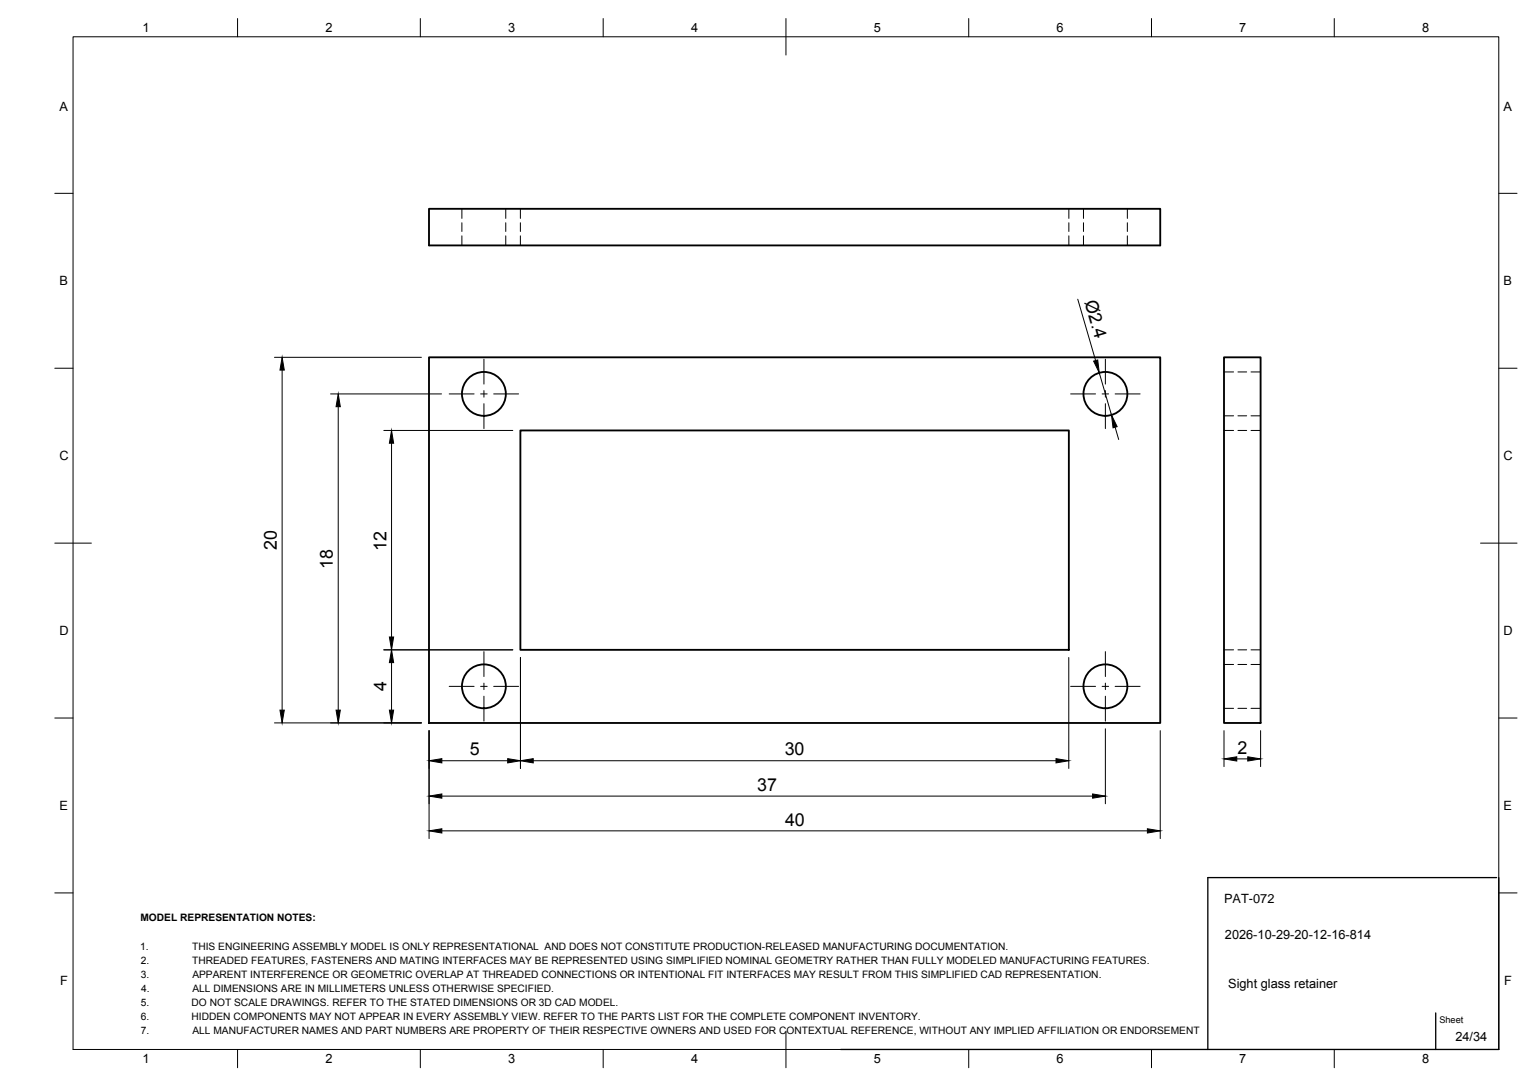
ISO-10303-21;
HEADER;
/* Generated by software containing ST-Developer
 * from STEP Tools, Inc. (www.steptools.com) 
 */

FILE_DESCRIPTION(
/* description */ ('PAT-072'),
/* implementation_level */ '2;1');

FILE_NAME(
/* name */ 'Sight glass retainer.step',
/* time_stamp */ '2026-10-29T20:11:56-07:00',
/* author */ (''),
/* organization */ (''),
/* preprocessor_version */ 'ST-DEVELOPER v20.2',
/* originating_system */ 'Autodesk Translation Framework v15.17.0.0',
/* authorisation */ '');

FILE_SCHEMA (('AUTOMOTIVE_DESIGN { 1 0 10303 214 3 1 1 }'));
ENDSEC;

DATA;
#10=MECHANICAL_DESIGN_GEOMETRIC_PRESENTATION_REPRESENTATION('',(#353),#11432);
#281=SHAPE_REPRESENTATION_RELATIONSHIP('SRR','None',#11585,#317);
#317=ADVANCED_BREP_SHAPE_REPRESENTATION('',(#389),#11416);
#353=STYLED_ITEM('',(#11812),#389);
#389=MANIFOLD_SOLID_BREP('Body1',#6088);
#518=FACE_BOUND('',#1510,.T.);
#519=FACE_BOUND('',#1511,.T.);
#520=FACE_BOUND('',#1512,.T.);
#521=FACE_BOUND('',#1513,.T.);
#522=FACE_BOUND('',#1514,.T.);
#523=FACE_BOUND('',#1517,.T.);
#524=FACE_BOUND('',#1518,.T.);
#525=FACE_BOUND('',#1519,.T.);
#526=FACE_BOUND('',#1520,.T.);
#527=FACE_BOUND('',#1521,.T.);
#692=PLANE('',#6942);
#693=PLANE('',#6943);
#694=PLANE('',#6944);
#695=PLANE('',#6945);
#696=PLANE('',#6946);
#697=PLANE('',#6947);
#698=PLANE('',#6948);
#699=PLANE('',#6949);
#700=PLANE('',#6950);
#701=PLANE('',#6951);
#1013=FACE_OUTER_BOUND('',#1501,.T.);
#1014=FACE_OUTER_BOUND('',#1502,.T.);
#1015=FACE_OUTER_BOUND('',#1503,.T.);
#1016=FACE_OUTER_BOUND('',#1504,.T.);
#1017=FACE_OUTER_BOUND('',#1505,.T.);
#1018=FACE_OUTER_BOUND('',#1506,.T.);
#1019=FACE_OUTER_BOUND('',#1507,.T.);
#1020=FACE_OUTER_BOUND('',#1508,.T.);
#1021=FACE_OUTER_BOUND('',#1509,.T.);
#1022=FACE_OUTER_BOUND('',#1515,.T.);
#1023=FACE_OUTER_BOUND('',#1516,.T.);
#1024=FACE_OUTER_BOUND('',#1522,.T.);
#1025=FACE_OUTER_BOUND('',#1523,.T.);
#1026=FACE_OUTER_BOUND('',#1524,.T.);
#1501=EDGE_LOOP('',(#4934,#4935,#4936,#4937));
#1502=EDGE_LOOP('',(#4938,#4939,#4940,#4941));
#1503=EDGE_LOOP('',(#4942,#4943,#4944,#4945));
#1504=EDGE_LOOP('',(#4946,#4947,#4948,#4949));
#1505=EDGE_LOOP('',(#4950,#4951,#4952,#4953));
#1506=EDGE_LOOP('',(#4954,#4955,#4956,#4957));
#1507=EDGE_LOOP('',(#4958,#4959,#4960,#4961));
#1508=EDGE_LOOP('',(#4962,#4963,#4964,#4965));
#1509=EDGE_LOOP('',(#4966,#4967,#4968,#4969));
#1510=EDGE_LOOP('',(#4970,#4971,#4972,#4973));
#1511=EDGE_LOOP('',(#4974));
#1512=EDGE_LOOP('',(#4975));
#1513=EDGE_LOOP('',(#4976));
#1514=EDGE_LOOP('',(#4977));
#1515=EDGE_LOOP('',(#4978,#4979,#4980,#4981));
#1516=EDGE_LOOP('',(#4982,#4983,#4984,#4985));
#1517=EDGE_LOOP('',(#4986,#4987,#4988,#4989));
#1518=EDGE_LOOP('',(#4990));
#1519=EDGE_LOOP('',(#4991));
#1520=EDGE_LOOP('',(#4992));
#1521=EDGE_LOOP('',(#4993));
#1522=EDGE_LOOP('',(#4994,#4995,#4996,#4997));
#1523=EDGE_LOOP('',(#4998,#4999,#5000,#5001));
#1524=EDGE_LOOP('',(#5002,#5003,#5004,#5005));
#1924=LINE('',#10622,#2343);
#1925=LINE('',#10628,#2344);
#1926=LINE('',#10634,#2345);
#1927=LINE('',#10640,#2346);
#1928=LINE('',#10645,#2347);
#1929=LINE('',#10647,#2348);
#1930=LINE('',#10649,#2349);
#1931=LINE('',#10650,#2350);
#1932=LINE('',#10653,#2351);
#1933=LINE('',#10655,#2352);
#1934=LINE('',#10656,#2353);
#1935=LINE('',#10659,#2354);
#1936=LINE('',#10661,#2355);
#1937=LINE('',#10662,#2356);
#1938=LINE('',#10664,#2357);
#1939=LINE('',#10665,#2358);
#1940=LINE('',#10669,#2359);
#1941=LINE('',#10671,#2360);
#1942=LINE('',#10673,#2361);
#1943=LINE('',#10674,#2362);
#1944=LINE('',#10677,#2363);
#1945=LINE('',#10679,#2364);
#1946=LINE('',#10680,#2365);
#1947=LINE('',#10683,#2366);
#1948=LINE('',#10685,#2367);
#1949=LINE('',#10686,#2368);
#1950=LINE('',#10688,#2369);
#1951=LINE('',#10689,#2370);
#2343=VECTOR('',#8335,0.12);
#2344=VECTOR('',#8342,0.12);
#2345=VECTOR('',#8349,0.12);
#2346=VECTOR('',#8356,0.12);
#2347=VECTOR('',#8361,1.);
#2348=VECTOR('',#8362,1.);
#2349=VECTOR('',#8363,1.);
#2350=VECTOR('',#8364,1.);
#2351=VECTOR('',#8367,1.);
#2352=VECTOR('',#8368,1.);
#2353=VECTOR('',#8369,1.);
#2354=VECTOR('',#8372,1.);
#2355=VECTOR('',#8373,1.);
#2356=VECTOR('',#8374,1.);
#2357=VECTOR('',#8377,1.);
#2358=VECTOR('',#8378,1.);
#2359=VECTOR('',#8381,1.);
#2360=VECTOR('',#8382,1.);
#2361=VECTOR('',#8383,1.);
#2362=VECTOR('',#8384,1.);
#2363=VECTOR('',#8387,1.);
#2364=VECTOR('',#8388,1.);
#2365=VECTOR('',#8389,1.);
#2366=VECTOR('',#8392,1.);
#2367=VECTOR('',#8393,1.);
#2368=VECTOR('',#8394,1.);
#2369=VECTOR('',#8397,1.);
#2370=VECTOR('',#8398,1.);
#2727=CIRCLE('',#6931,0.12);
#2728=CIRCLE('',#6932,0.12);
#2729=CIRCLE('',#6934,0.12);
#2730=CIRCLE('',#6935,0.12);
#2731=CIRCLE('',#6937,0.12);
#2732=CIRCLE('',#6938,0.12);
#2733=CIRCLE('',#6940,0.12);
#2734=CIRCLE('',#6941,0.12);
#3118=VERTEX_POINT('',#10619);
#3119=VERTEX_POINT('',#10621);
#3120=VERTEX_POINT('',#10625);
#3121=VERTEX_POINT('',#10627);
#3122=VERTEX_POINT('',#10631);
#3123=VERTEX_POINT('',#10633);
#3124=VERTEX_POINT('',#10637);
#3125=VERTEX_POINT('',#10639);
#3126=VERTEX_POINT('',#10643);
#3127=VERTEX_POINT('',#10644);
#3128=VERTEX_POINT('',#10646);
#3129=VERTEX_POINT('',#10648);
#3130=VERTEX_POINT('',#10652);
#3131=VERTEX_POINT('',#10654);
#3132=VERTEX_POINT('',#10658);
#3133=VERTEX_POINT('',#10660);
#3134=VERTEX_POINT('',#10667);
#3135=VERTEX_POINT('',#10668);
#3136=VERTEX_POINT('',#10670);
#3137=VERTEX_POINT('',#10672);
#3138=VERTEX_POINT('',#10676);
#3139=VERTEX_POINT('',#10678);
#3140=VERTEX_POINT('',#10682);
#3141=VERTEX_POINT('',#10684);
#3756=EDGE_CURVE('',#3118,#3118,#2727,.T.);
#3757=EDGE_CURVE('',#3118,#3119,#1924,.T.);
#3758=EDGE_CURVE('',#3119,#3119,#2728,.T.);
#3759=EDGE_CURVE('',#3120,#3120,#2729,.T.);
#3760=EDGE_CURVE('',#3120,#3121,#1925,.T.);
#3761=EDGE_CURVE('',#3121,#3121,#2730,.T.);
#3762=EDGE_CURVE('',#3122,#3122,#2731,.T.);
#3763=EDGE_CURVE('',#3122,#3123,#1926,.T.);
#3764=EDGE_CURVE('',#3123,#3123,#2732,.T.);
#3765=EDGE_CURVE('',#3124,#3124,#2733,.T.);
#3766=EDGE_CURVE('',#3124,#3125,#1927,.T.);
#3767=EDGE_CURVE('',#3125,#3125,#2734,.T.);
#3768=EDGE_CURVE('',#3126,#3127,#1928,.T.);
#3769=EDGE_CURVE('',#3128,#3126,#1929,.T.);
#3770=EDGE_CURVE('',#3129,#3128,#1930,.T.);
#3771=EDGE_CURVE('',#3129,#3127,#1931,.T.);
#3772=EDGE_CURVE('',#3127,#3130,#1932,.T.);
#3773=EDGE_CURVE('',#3131,#3129,#1933,.T.);
#3774=EDGE_CURVE('',#3131,#3130,#1934,.T.);
#3775=EDGE_CURVE('',#3130,#3132,#1935,.T.);
#3776=EDGE_CURVE('',#3133,#3131,#1936,.T.);
#3777=EDGE_CURVE('',#3133,#3132,#1937,.T.);
#3778=EDGE_CURVE('',#3132,#3126,#1938,.T.);
#3779=EDGE_CURVE('',#3128,#3133,#1939,.T.);
#3780=EDGE_CURVE('',#3134,#3135,#1940,.T.);
#3781=EDGE_CURVE('',#3135,#3136,#1941,.T.);
#3782=EDGE_CURVE('',#3137,#3136,#1942,.T.);
#3783=EDGE_CURVE('',#3134,#3137,#1943,.T.);
#3784=EDGE_CURVE('',#3138,#3134,#1944,.T.);
#3785=EDGE_CURVE('',#3139,#3137,#1945,.T.);
#3786=EDGE_CURVE('',#3138,#3139,#1946,.T.);
#3787=EDGE_CURVE('',#3140,#3138,#1947,.T.);
#3788=EDGE_CURVE('',#3141,#3139,#1948,.T.);
#3789=EDGE_CURVE('',#3140,#3141,#1949,.T.);
#3790=EDGE_CURVE('',#3135,#3140,#1950,.T.);
#3791=EDGE_CURVE('',#3136,#3141,#1951,.T.);
#4934=ORIENTED_EDGE('',*,*,#3756,.F.);
#4935=ORIENTED_EDGE('',*,*,#3757,.T.);
#4936=ORIENTED_EDGE('',*,*,#3758,.F.);
#4937=ORIENTED_EDGE('',*,*,#3757,.F.);
#4938=ORIENTED_EDGE('',*,*,#3759,.F.);
#4939=ORIENTED_EDGE('',*,*,#3760,.T.);
#4940=ORIENTED_EDGE('',*,*,#3761,.F.);
#4941=ORIENTED_EDGE('',*,*,#3760,.F.);
#4942=ORIENTED_EDGE('',*,*,#3762,.F.);
#4943=ORIENTED_EDGE('',*,*,#3763,.T.);
#4944=ORIENTED_EDGE('',*,*,#3764,.F.);
#4945=ORIENTED_EDGE('',*,*,#3763,.F.);
#4946=ORIENTED_EDGE('',*,*,#3765,.F.);
#4947=ORIENTED_EDGE('',*,*,#3766,.T.);
#4948=ORIENTED_EDGE('',*,*,#3767,.F.);
#4949=ORIENTED_EDGE('',*,*,#3766,.F.);
#4950=ORIENTED_EDGE('',*,*,#3768,.F.);
#4951=ORIENTED_EDGE('',*,*,#3769,.F.);
#4952=ORIENTED_EDGE('',*,*,#3770,.F.);
#4953=ORIENTED_EDGE('',*,*,#3771,.T.);
#4954=ORIENTED_EDGE('',*,*,#3772,.F.);
#4955=ORIENTED_EDGE('',*,*,#3771,.F.);
#4956=ORIENTED_EDGE('',*,*,#3773,.F.);
#4957=ORIENTED_EDGE('',*,*,#3774,.T.);
#4958=ORIENTED_EDGE('',*,*,#3775,.F.);
#4959=ORIENTED_EDGE('',*,*,#3774,.F.);
#4960=ORIENTED_EDGE('',*,*,#3776,.F.);
#4961=ORIENTED_EDGE('',*,*,#3777,.T.);
#4962=ORIENTED_EDGE('',*,*,#3778,.F.);
#4963=ORIENTED_EDGE('',*,*,#3777,.F.);
#4964=ORIENTED_EDGE('',*,*,#3779,.F.);
#4965=ORIENTED_EDGE('',*,*,#3769,.T.);
#4966=ORIENTED_EDGE('',*,*,#3780,.T.);
#4967=ORIENTED_EDGE('',*,*,#3781,.T.);
#4968=ORIENTED_EDGE('',*,*,#3782,.F.);
#4969=ORIENTED_EDGE('',*,*,#3783,.F.);
#4970=ORIENTED_EDGE('',*,*,#3775,.T.);
#4971=ORIENTED_EDGE('',*,*,#3778,.T.);
#4972=ORIENTED_EDGE('',*,*,#3768,.T.);
#4973=ORIENTED_EDGE('',*,*,#3772,.T.);
#4974=ORIENTED_EDGE('',*,*,#3767,.T.);
#4975=ORIENTED_EDGE('',*,*,#3764,.T.);
#4976=ORIENTED_EDGE('',*,*,#3761,.T.);
#4977=ORIENTED_EDGE('',*,*,#3758,.T.);
#4978=ORIENTED_EDGE('',*,*,#3784,.T.);
#4979=ORIENTED_EDGE('',*,*,#3783,.T.);
#4980=ORIENTED_EDGE('',*,*,#3785,.F.);
#4981=ORIENTED_EDGE('',*,*,#3786,.F.);
#4982=ORIENTED_EDGE('',*,*,#3787,.T.);
#4983=ORIENTED_EDGE('',*,*,#3786,.T.);
#4984=ORIENTED_EDGE('',*,*,#3788,.F.);
#4985=ORIENTED_EDGE('',*,*,#3789,.F.);
#4986=ORIENTED_EDGE('',*,*,#3776,.T.);
#4987=ORIENTED_EDGE('',*,*,#3773,.T.);
#4988=ORIENTED_EDGE('',*,*,#3770,.T.);
#4989=ORIENTED_EDGE('',*,*,#3779,.T.);
#4990=ORIENTED_EDGE('',*,*,#3765,.T.);
#4991=ORIENTED_EDGE('',*,*,#3762,.T.);
#4992=ORIENTED_EDGE('',*,*,#3759,.T.);
#4993=ORIENTED_EDGE('',*,*,#3756,.T.);
#4994=ORIENTED_EDGE('',*,*,#3790,.T.);
#4995=ORIENTED_EDGE('',*,*,#3789,.T.);
#4996=ORIENTED_EDGE('',*,*,#3791,.F.);
#4997=ORIENTED_EDGE('',*,*,#3781,.F.);
#4998=ORIENTED_EDGE('',*,*,#3791,.T.);
#4999=ORIENTED_EDGE('',*,*,#3788,.T.);
#5000=ORIENTED_EDGE('',*,*,#3785,.T.);
#5001=ORIENTED_EDGE('',*,*,#3782,.T.);
#5002=ORIENTED_EDGE('',*,*,#3790,.F.);
#5003=ORIENTED_EDGE('',*,*,#3780,.F.);
#5004=ORIENTED_EDGE('',*,*,#3784,.F.);
#5005=ORIENTED_EDGE('',*,*,#3787,.F.);
#5653=CYLINDRICAL_SURFACE('',#6930,0.12);
#5654=CYLINDRICAL_SURFACE('',#6933,0.12);
#5655=CYLINDRICAL_SURFACE('',#6936,0.12);
#5656=CYLINDRICAL_SURFACE('',#6939,0.12);
#5912=ADVANCED_FACE('',(#1013),#5653,.F.);
#5913=ADVANCED_FACE('',(#1014),#5654,.F.);
#5914=ADVANCED_FACE('',(#1015),#5655,.F.);
#5915=ADVANCED_FACE('',(#1016),#5656,.F.);
#5916=ADVANCED_FACE('',(#1017),#692,.F.);
#5917=ADVANCED_FACE('',(#1018),#693,.F.);
#5918=ADVANCED_FACE('',(#1019),#694,.F.);
#5919=ADVANCED_FACE('',(#1020),#695,.F.);
#5920=ADVANCED_FACE('',(#1021,#518,#519,#520,#521,#522),#696,.T.);
#5921=ADVANCED_FACE('',(#1022),#697,.T.);
#5922=ADVANCED_FACE('',(#1023,#523,#524,#525,#526,#527),#698,.T.);
#5923=ADVANCED_FACE('',(#1024),#699,.T.);
#5924=ADVANCED_FACE('',(#1025),#700,.T.);
#5925=ADVANCED_FACE('',(#1026),#701,.F.);
#6088=CLOSED_SHELL('',(#5912,#5913,#5914,#5915,#5916,#5917,#5918,#5919,
#5920,#5921,#5922,#5923,#5924,#5925));
#6929=AXIS2_PLACEMENT_3D('',#10617,#8329,#8330);
#6930=AXIS2_PLACEMENT_3D('',#10618,#8331,#8332);
#6931=AXIS2_PLACEMENT_3D('',#10620,#8333,#8334);
#6932=AXIS2_PLACEMENT_3D('',#10623,#8336,#8337);
#6933=AXIS2_PLACEMENT_3D('',#10624,#8338,#8339);
#6934=AXIS2_PLACEMENT_3D('',#10626,#8340,#8341);
#6935=AXIS2_PLACEMENT_3D('',#10629,#8343,#8344);
#6936=AXIS2_PLACEMENT_3D('',#10630,#8345,#8346);
#6937=AXIS2_PLACEMENT_3D('',#10632,#8347,#8348);
#6938=AXIS2_PLACEMENT_3D('',#10635,#8350,#8351);
#6939=AXIS2_PLACEMENT_3D('',#10636,#8352,#8353);
#6940=AXIS2_PLACEMENT_3D('',#10638,#8354,#8355);
#6941=AXIS2_PLACEMENT_3D('',#10641,#8357,#8358);
#6942=AXIS2_PLACEMENT_3D('',#10642,#8359,#8360);
#6943=AXIS2_PLACEMENT_3D('',#10651,#8365,#8366);
#6944=AXIS2_PLACEMENT_3D('',#10657,#8370,#8371);
#6945=AXIS2_PLACEMENT_3D('',#10663,#8375,#8376);
#6946=AXIS2_PLACEMENT_3D('',#10666,#8379,#8380);
#6947=AXIS2_PLACEMENT_3D('',#10675,#8385,#8386);
#6948=AXIS2_PLACEMENT_3D('',#10681,#8390,#8391);
#6949=AXIS2_PLACEMENT_3D('',#10687,#8395,#8396);
#6950=AXIS2_PLACEMENT_3D('',#10690,#8399,#8400);
#6951=AXIS2_PLACEMENT_3D('',#10691,#8401,#8402);
#8329=DIRECTION('axis',(0.,0.,1.));
#8330=DIRECTION('refdir',(1.,0.,0.));
#8331=DIRECTION('center_axis',(0.,1.,0.));
#8332=DIRECTION('ref_axis',(1.,0.,0.));
#8333=DIRECTION('center_axis',(0.,1.,0.));
#8334=DIRECTION('ref_axis',(1.,0.,0.));
#8335=DIRECTION('',(0.,1.,0.));
#8336=DIRECTION('center_axis',(0.,-1.,0.));
#8337=DIRECTION('ref_axis',(1.,0.,0.));
#8338=DIRECTION('center_axis',(0.,1.,0.));
#8339=DIRECTION('ref_axis',(1.,0.,0.));
#8340=DIRECTION('center_axis',(0.,1.,0.));
#8341=DIRECTION('ref_axis',(1.,0.,0.));
#8342=DIRECTION('',(0.,1.,0.));
#8343=DIRECTION('center_axis',(0.,-1.,0.));
#8344=DIRECTION('ref_axis',(1.,0.,0.));
#8345=DIRECTION('center_axis',(0.,1.,0.));
#8346=DIRECTION('ref_axis',(1.,0.,0.));
#8347=DIRECTION('center_axis',(0.,1.,0.));
#8348=DIRECTION('ref_axis',(1.,0.,0.));
#8349=DIRECTION('',(0.,1.,0.));
#8350=DIRECTION('center_axis',(0.,-1.,0.));
#8351=DIRECTION('ref_axis',(1.,0.,0.));
#8352=DIRECTION('center_axis',(0.,1.,0.));
#8353=DIRECTION('ref_axis',(1.,0.,0.));
#8354=DIRECTION('center_axis',(0.,1.,0.));
#8355=DIRECTION('ref_axis',(1.,0.,0.));
#8356=DIRECTION('',(0.,1.,0.));
#8357=DIRECTION('center_axis',(0.,-1.,0.));
#8358=DIRECTION('ref_axis',(1.,0.,0.));
#8359=DIRECTION('center_axis',(1.,0.,0.));
#8360=DIRECTION('ref_axis',(0.,0.,-1.));
#8361=DIRECTION('',(0.,0.,1.));
#8362=DIRECTION('',(0.,1.,0.));
#8363=DIRECTION('',(0.,0.,-1.));
#8364=DIRECTION('',(0.,1.,0.));
#8365=DIRECTION('center_axis',(0.,0.,1.));
#8366=DIRECTION('ref_axis',(1.,0.,0.));
#8367=DIRECTION('',(-1.,0.,0.));
#8368=DIRECTION('',(1.,0.,0.));
#8369=DIRECTION('',(0.,1.,0.));
#8370=DIRECTION('center_axis',(-1.,0.,0.));
#8371=DIRECTION('ref_axis',(0.,0.,1.));
#8372=DIRECTION('',(0.,0.,-1.));
#8373=DIRECTION('',(0.,0.,1.));
#8374=DIRECTION('',(0.,1.,0.));
#8375=DIRECTION('center_axis',(0.,0.,-1.));
#8376=DIRECTION('ref_axis',(-1.,0.,0.));
#8377=DIRECTION('',(1.,0.,0.));
#8378=DIRECTION('',(-1.,0.,0.));
#8379=DIRECTION('center_axis',(0.,1.,0.));
#8380=DIRECTION('ref_axis',(-1.,0.,0.));
#8381=DIRECTION('',(-1.,0.,0.));
#8382=DIRECTION('',(0.,0.,1.));
#8383=DIRECTION('',(-1.,0.,0.));
#8384=DIRECTION('',(0.,0.,1.));
#8385=DIRECTION('center_axis',(1.,0.,0.));
#8386=DIRECTION('ref_axis',(0.,1.,0.));
#8387=DIRECTION('',(0.,1.,0.));
#8388=DIRECTION('',(0.,1.,0.));
#8389=DIRECTION('',(0.,0.,1.));
#8390=DIRECTION('center_axis',(0.,-1.,0.));
#8391=DIRECTION('ref_axis',(1.,0.,0.));
#8392=DIRECTION('',(1.,0.,0.));
#8393=DIRECTION('',(1.,0.,0.));
#8394=DIRECTION('',(0.,0.,1.));
#8395=DIRECTION('center_axis',(-1.,0.,0.));
#8396=DIRECTION('ref_axis',(0.,-1.,0.));
#8397=DIRECTION('',(0.,-1.,0.));
#8398=DIRECTION('',(0.,-1.,0.));
#8399=DIRECTION('center_axis',(0.,0.,1.));
#8400=DIRECTION('ref_axis',(1.,0.,0.));
#8401=DIRECTION('center_axis',(0.,0.,1.));
#8402=DIRECTION('ref_axis',(1.,0.,0.));
#10617=CARTESIAN_POINT('',(0.,0.,0.));
#10618=CARTESIAN_POINT('Origin',(0.8,-3.2,9.8));
#10619=CARTESIAN_POINT('',(0.68,-3.1,9.8));
#10620=CARTESIAN_POINT('Origin',(0.8,-3.1,9.8));
#10621=CARTESIAN_POINT('',(0.68,-2.9,9.8));
#10622=CARTESIAN_POINT('',(0.68,-3.2,9.8));
#10623=CARTESIAN_POINT('Origin',(0.8,-2.9,9.8));
#10624=CARTESIAN_POINT('Origin',(-0.8,-3.2,13.2));
#10625=CARTESIAN_POINT('',(-0.92,-3.1,13.2));
#10626=CARTESIAN_POINT('Origin',(-0.8,-3.1,13.2));
#10627=CARTESIAN_POINT('',(-0.92,-2.9,13.2));
#10628=CARTESIAN_POINT('',(-0.92,-3.2,13.2));
#10629=CARTESIAN_POINT('Origin',(-0.8,-2.9,13.2));
#10630=CARTESIAN_POINT('Origin',(-0.8,-3.2,9.8));
#10631=CARTESIAN_POINT('',(-0.92,-3.1,9.8));
#10632=CARTESIAN_POINT('Origin',(-0.8,-3.1,9.8));
#10633=CARTESIAN_POINT('',(-0.92,-2.9,9.8));
#10634=CARTESIAN_POINT('',(-0.92,-3.2,9.8));
#10635=CARTESIAN_POINT('Origin',(-0.8,-2.9,9.8));
#10636=CARTESIAN_POINT('Origin',(0.8,-3.2,13.2));
#10637=CARTESIAN_POINT('',(0.68,-3.1,13.2));
#10638=CARTESIAN_POINT('Origin',(0.8,-3.1,13.2));
#10639=CARTESIAN_POINT('',(0.68,-2.9,13.2));
#10640=CARTESIAN_POINT('',(0.68,-3.2,13.2));
#10641=CARTESIAN_POINT('Origin',(0.8,-2.9,13.2));
#10642=CARTESIAN_POINT('Origin',(0.6,-3.2,13.));
#10643=CARTESIAN_POINT('',(0.6,-2.9,10.));
#10644=CARTESIAN_POINT('',(0.6,-2.9,13.));
#10645=CARTESIAN_POINT('',(0.6,-2.9,11.25));
#10646=CARTESIAN_POINT('',(0.6,-3.1,10.));
#10647=CARTESIAN_POINT('',(0.6,-3.2,10.));
#10648=CARTESIAN_POINT('',(0.6,-3.1,13.));
#10649=CARTESIAN_POINT('',(0.6,-3.1,11.25));
#10650=CARTESIAN_POINT('',(0.6,-3.2,13.));
#10651=CARTESIAN_POINT('Origin',(-0.6,-3.2,13.));
#10652=CARTESIAN_POINT('',(-0.6,-2.9,13.));
#10653=CARTESIAN_POINT('',(0.2,-2.9,13.));
#10654=CARTESIAN_POINT('',(-0.6,-3.1,13.));
#10655=CARTESIAN_POINT('',(-0.8,-3.1,13.));
#10656=CARTESIAN_POINT('',(-0.6,-3.2,13.));
#10657=CARTESIAN_POINT('Origin',(-0.6,-3.2,10.));
#10658=CARTESIAN_POINT('',(-0.6,-2.9,10.));
#10659=CARTESIAN_POINT('',(-0.6,-2.9,9.75));
#10660=CARTESIAN_POINT('',(-0.6,-3.1,10.));
#10661=CARTESIAN_POINT('',(-0.6,-3.1,9.75));
#10662=CARTESIAN_POINT('',(-0.6,-3.2,10.));
#10663=CARTESIAN_POINT('Origin',(0.6,-3.2,10.));
#10664=CARTESIAN_POINT('',(0.8,-2.9,10.));
#10665=CARTESIAN_POINT('',(-0.2,-3.1,10.));
#10666=CARTESIAN_POINT('Origin',(1.,-2.9,9.5));
#10667=CARTESIAN_POINT('',(1.,-2.9,9.5));
#10668=CARTESIAN_POINT('',(-1.,-2.9,9.5));
#10669=CARTESIAN_POINT('',(1.,-2.9,9.5));
#10670=CARTESIAN_POINT('',(-1.,-2.9,13.5));
#10671=CARTESIAN_POINT('',(-1.,-2.9,9.5));
#10672=CARTESIAN_POINT('',(1.,-2.9,13.5));
#10673=CARTESIAN_POINT('',(1.,-2.9,13.5));
#10674=CARTESIAN_POINT('',(1.,-2.9,9.5));
#10675=CARTESIAN_POINT('Origin',(1.,-3.1,9.5));
#10676=CARTESIAN_POINT('',(1.,-3.1,9.5));
#10677=CARTESIAN_POINT('',(1.,-3.1,9.5));
#10678=CARTESIAN_POINT('',(1.,-3.1,13.5));
#10679=CARTESIAN_POINT('',(1.,-3.1,13.5));
#10680=CARTESIAN_POINT('',(1.,-3.1,9.5));
#10681=CARTESIAN_POINT('Origin',(-1.,-3.1,9.5));
#10682=CARTESIAN_POINT('',(-1.,-3.1,9.5));
#10683=CARTESIAN_POINT('',(-1.,-3.1,9.5));
#10684=CARTESIAN_POINT('',(-1.,-3.1,13.5));
#10685=CARTESIAN_POINT('',(-1.,-3.1,13.5));
#10686=CARTESIAN_POINT('',(-1.,-3.1,9.5));
#10687=CARTESIAN_POINT('Origin',(-1.,-2.9,9.5));
#10688=CARTESIAN_POINT('',(-1.,-2.9,9.5));
#10689=CARTESIAN_POINT('',(-1.,-2.9,13.5));
#10690=CARTESIAN_POINT('Origin',(0.,-3.,13.5));
#10691=CARTESIAN_POINT('Origin',(0.,-3.,9.5));
#11377=UNCERTAINTY_MEASURE_WITH_UNIT(LENGTH_MEASURE(0.001),#11433,
'DISTANCE_ACCURACY_VALUE',
'Maximum model space distance between geometric entities at asserted c
onnectivities');
#11393=UNCERTAINTY_MEASURE_WITH_UNIT(LENGTH_MEASURE(0.001),#11433,
'DISTANCE_ACCURACY_VALUE',
'Maximum model space distance between geometric entities at asserted c
onnectivities');
#11416=(
GEOMETRIC_REPRESENTATION_CONTEXT(3)
GLOBAL_UNCERTAINTY_ASSIGNED_CONTEXT((#11377))
GLOBAL_UNIT_ASSIGNED_CONTEXT((#11433,#11435,#11436))
REPRESENTATION_CONTEXT('','3D')
);
#11432=(
GEOMETRIC_REPRESENTATION_CONTEXT(3)
GLOBAL_UNCERTAINTY_ASSIGNED_CONTEXT((#11393))
GLOBAL_UNIT_ASSIGNED_CONTEXT((#11433,#11435,#11436))
REPRESENTATION_CONTEXT('','3D')
);
#11433=(
LENGTH_UNIT()
NAMED_UNIT(*)
SI_UNIT(.CENTI.,.METRE.)
);
#11435=(
NAMED_UNIT(*)
PLANE_ANGLE_UNIT()
SI_UNIT($,.RADIAN.)
);
#11436=(
NAMED_UNIT(*)
SI_UNIT($,.STERADIAN.)
SOLID_ANGLE_UNIT()
);
#11459=SHAPE_DEFINITION_REPRESENTATION(#11497,#11585);
#11497=PRODUCT_DEFINITION_SHAPE('',$,#11624);
#11585=SHAPE_REPRESENTATION('',(#6929),#11416);
#11601=PRODUCT_DEFINITION_CONTEXT('part definition',#11717,'design');
#11624=PRODUCT_DEFINITION('Sight glass retainer',
'Sight glass retainer',#11662,#11601);
#11662=PRODUCT_DEFINITION_FORMATION('',$,#11741);
#11717=APPLICATION_CONTEXT(
'Core Data for Automotive Mechanical Design Process');
#11718=PRODUCT_CONTEXT('part definition',#11717,'mechanical');
#11741=PRODUCT('Sight glass retainer','Sight glass retainer',
'Sight glass retainer',(#11718));
#11806=COLOUR_RGB('Sky Blue',0.24,0.69,0.87);
#11807=FILL_AREA_STYLE_COLOUR('',#11806);
#11808=FILL_AREA_STYLE('',(#11807));
#11809=SURFACE_STYLE_FILL_AREA(#11808);
#11810=SURFACE_SIDE_STYLE('',(#11809));
#11811=SURFACE_STYLE_USAGE(.BOTH.,#11810);
#11812=PRESENTATION_STYLE_ASSIGNMENT((#11811));
ENDSEC;
END-ISO-10303-21;
